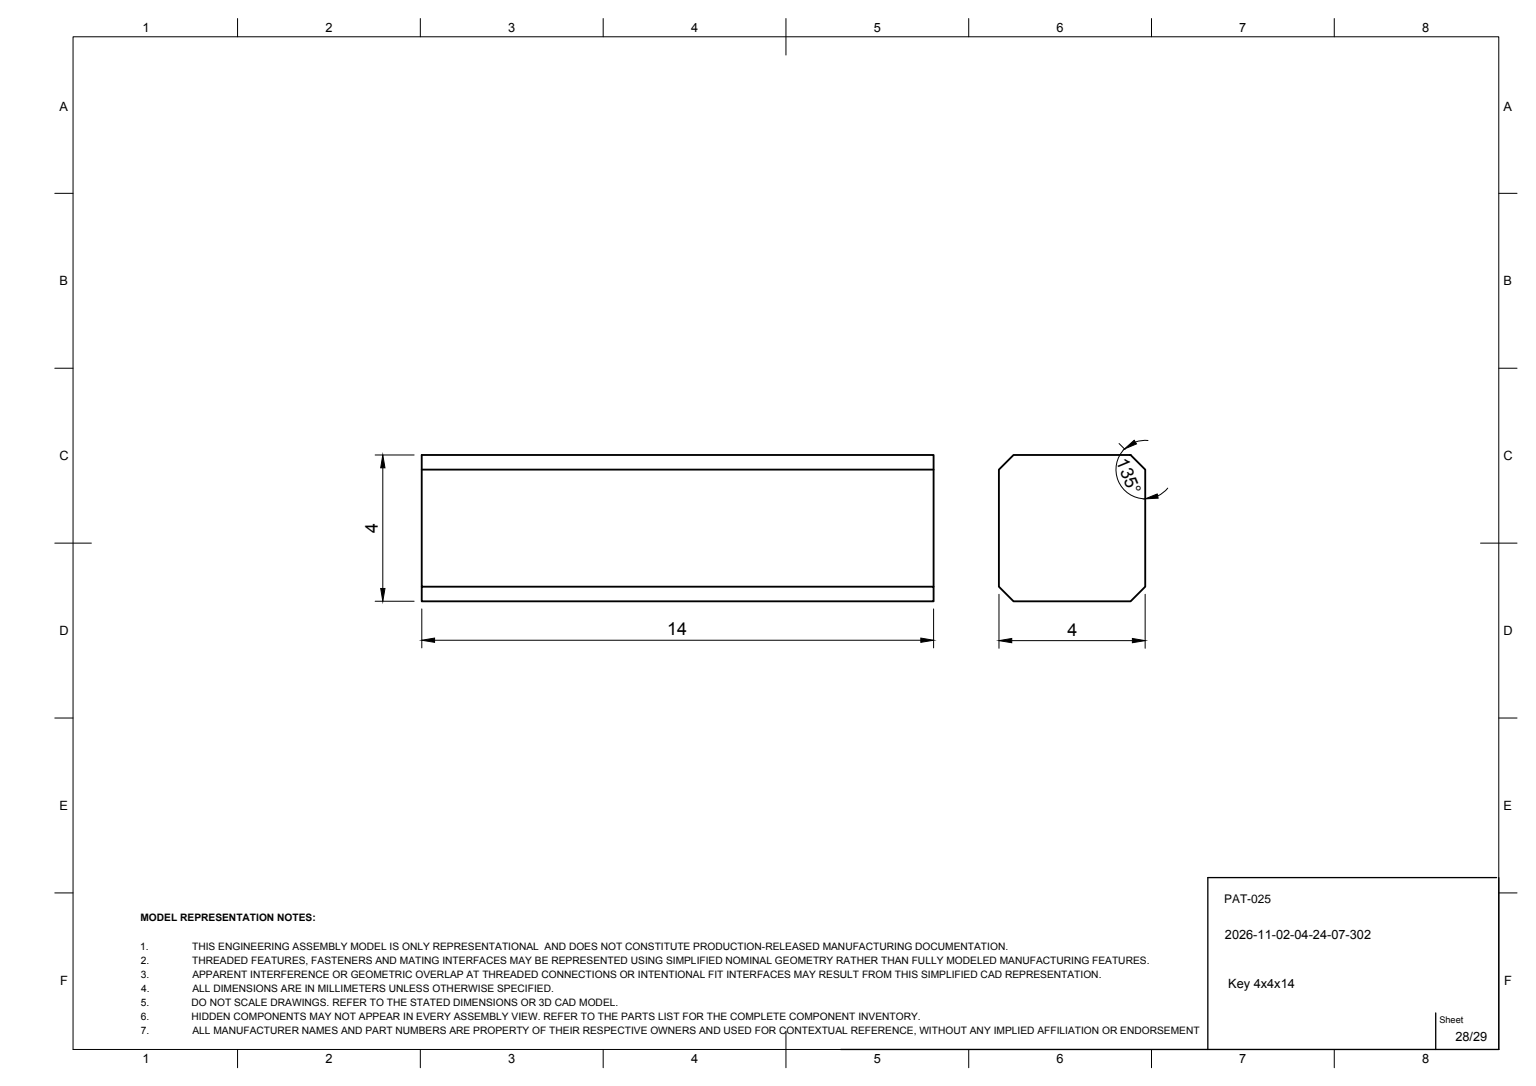
ISO-10303-21;
HEADER;
/* Generated by software containing ST-Developer
 * from STEP Tools, Inc. (www.steptools.com) 
 */

FILE_DESCRIPTION(
/* description */ ('Counter shaft with two pulleys and keyed hub'),
/* implementation_level */ '2;1');

FILE_NAME(
/* name */ 'Key 4x4x14.step',
/* time_stamp */ '2026-10-27T10:46:10-07:00',
/* author */ (''),
/* organization */ (''),
/* preprocessor_version */ 'ST-DEVELOPER v20.2',
/* originating_system */ 'Autodesk Translation Framework v15.17.0.0',
/* authorisation */ '');

FILE_SCHEMA (('AUTOMOTIVE_DESIGN { 1 0 10303 214 3 1 1 }'));
ENDSEC;

DATA;
#10=MECHANICAL_DESIGN_GEOMETRIC_PRESENTATION_REPRESENTATION('',(#312),#10821);
#261=SHAPE_REPRESENTATION_RELATIONSHIP('SRR','None',#10949,#286);
#286=ADVANCED_BREP_SHAPE_REPRESENTATION('',(#337),#10817);
#312=STYLED_ITEM('',(#11135),#337);
#337=MANIFOLD_SOLID_BREP('Body1',#5596);
#548=PLANE('',#6474);
#549=PLANE('',#6475);
#550=PLANE('',#6476);
#551=PLANE('',#6477);
#552=PLANE('',#6478);
#553=PLANE('',#6479);
#554=PLANE('',#6480);
#555=PLANE('',#6481);
#556=PLANE('',#6482);
#557=PLANE('',#6483);
#853=FACE_OUTER_BOUND('',#1256,.T.);
#854=FACE_OUTER_BOUND('',#1257,.T.);
#855=FACE_OUTER_BOUND('',#1258,.T.);
#856=FACE_OUTER_BOUND('',#1259,.T.);
#857=FACE_OUTER_BOUND('',#1260,.T.);
#858=FACE_OUTER_BOUND('',#1261,.T.);
#859=FACE_OUTER_BOUND('',#1262,.T.);
#860=FACE_OUTER_BOUND('',#1263,.T.);
#861=FACE_OUTER_BOUND('',#1264,.T.);
#862=FACE_OUTER_BOUND('',#1265,.T.);
#1256=EDGE_LOOP('',(#4903,#4904,#4905,#4906,#4907,#4908,#4909,#4910));
#1257=EDGE_LOOP('',(#4911,#4912,#4913,#4914));
#1258=EDGE_LOOP('',(#4915,#4916,#4917,#4918));
#1259=EDGE_LOOP('',(#4919,#4920,#4921,#4922));
#1260=EDGE_LOOP('',(#4923,#4924,#4925,#4926));
#1261=EDGE_LOOP('',(#4927,#4928,#4929,#4930,#4931,#4932,#4933,#4934));
#1262=EDGE_LOOP('',(#4935,#4936,#4937,#4938));
#1263=EDGE_LOOP('',(#4939,#4940,#4941,#4942));
#1264=EDGE_LOOP('',(#4943,#4944,#4945,#4946));
#1265=EDGE_LOOP('',(#4947,#4948,#4949,#4950));
#1603=LINE('',#10519,#1992);
#1604=LINE('',#10521,#1993);
#1605=LINE('',#10523,#1994);
#1606=LINE('',#10525,#1995);
#1607=LINE('',#10527,#1996);
#1608=LINE('',#10529,#1997);
#1609=LINE('',#10531,#1998);
#1610=LINE('',#10532,#1999);
#1611=LINE('',#10535,#2000);
#1612=LINE('',#10537,#2001);
#1613=LINE('',#10538,#2002);
#1614=LINE('',#10541,#2003);
#1615=LINE('',#10542,#2004);
#1616=LINE('',#10545,#2005);
#1617=LINE('',#10546,#2006);
#1618=LINE('',#10549,#2007);
#1619=LINE('',#10550,#2008);
#1620=LINE('',#10553,#2009);
#1621=LINE('',#10555,#2010);
#1622=LINE('',#10557,#2011);
#1623=LINE('',#10558,#2012);
#1624=LINE('',#10560,#2013);
#1625=LINE('',#10562,#2014);
#1626=LINE('',#10564,#2015);
#1992=VECTOR('',#8051,1.);
#1993=VECTOR('',#8052,1.);
#1994=VECTOR('',#8053,1.);
#1995=VECTOR('',#8054,1.);
#1996=VECTOR('',#8055,1.);
#1997=VECTOR('',#8056,1.);
#1998=VECTOR('',#8057,1.);
#1999=VECTOR('',#8058,1.);
#2000=VECTOR('',#8061,1.);
#2001=VECTOR('',#8062,1.);
#2002=VECTOR('',#8063,1.);
#2003=VECTOR('',#8066,1.);
#2004=VECTOR('',#8067,1.);
#2005=VECTOR('',#8070,1.);
#2006=VECTOR('',#8071,1.);
#2007=VECTOR('',#8074,1.);
#2008=VECTOR('',#8075,1.);
#2009=VECTOR('',#8078,1.);
#2010=VECTOR('',#8079,1.);
#2011=VECTOR('',#8080,1.);
#2012=VECTOR('',#8081,1.);
#2013=VECTOR('',#8084,1.);
#2014=VECTOR('',#8087,1.);
#2015=VECTOR('',#8090,1.);
#2819=VERTEX_POINT('',#10517);
#2820=VERTEX_POINT('',#10518);
#2821=VERTEX_POINT('',#10520);
#2822=VERTEX_POINT('',#10522);
#2823=VERTEX_POINT('',#10524);
#2824=VERTEX_POINT('',#10526);
#2825=VERTEX_POINT('',#10528);
#2826=VERTEX_POINT('',#10530);
#2827=VERTEX_POINT('',#10534);
#2828=VERTEX_POINT('',#10536);
#2829=VERTEX_POINT('',#10540);
#2830=VERTEX_POINT('',#10544);
#2831=VERTEX_POINT('',#10548);
#2832=VERTEX_POINT('',#10552);
#2833=VERTEX_POINT('',#10554);
#2834=VERTEX_POINT('',#10556);
#3524=EDGE_CURVE('',#2819,#2820,#1603,.T.);
#3525=EDGE_CURVE('',#2821,#2819,#1604,.T.);
#3526=EDGE_CURVE('',#2822,#2821,#1605,.T.);
#3527=EDGE_CURVE('',#2823,#2822,#1606,.T.);
#3528=EDGE_CURVE('',#2824,#2823,#1607,.T.);
#3529=EDGE_CURVE('',#2825,#2824,#1608,.T.);
#3530=EDGE_CURVE('',#2826,#2825,#1609,.T.);
#3531=EDGE_CURVE('',#2820,#2826,#1610,.T.);
#3532=EDGE_CURVE('',#2823,#2827,#1611,.T.);
#3533=EDGE_CURVE('',#2827,#2828,#1612,.T.);
#3534=EDGE_CURVE('',#2828,#2824,#1613,.T.);
#3535=EDGE_CURVE('',#2829,#2822,#1614,.T.);
#3536=EDGE_CURVE('',#2829,#2827,#1615,.T.);
#3537=EDGE_CURVE('',#2821,#2830,#1616,.T.);
#3538=EDGE_CURVE('',#2830,#2829,#1617,.T.);
#3539=EDGE_CURVE('',#2831,#2819,#1618,.T.);
#3540=EDGE_CURVE('',#2831,#2830,#1619,.T.);
#3541=EDGE_CURVE('',#2832,#2831,#1620,.T.);
#3542=EDGE_CURVE('',#2833,#2832,#1621,.T.);
#3543=EDGE_CURVE('',#2834,#2833,#1622,.T.);
#3544=EDGE_CURVE('',#2828,#2834,#1623,.T.);
#3545=EDGE_CURVE('',#2820,#2832,#1624,.T.);
#3546=EDGE_CURVE('',#2833,#2826,#1625,.T.);
#3547=EDGE_CURVE('',#2825,#2834,#1626,.T.);
#4903=ORIENTED_EDGE('',*,*,#3524,.F.);
#4904=ORIENTED_EDGE('',*,*,#3525,.F.);
#4905=ORIENTED_EDGE('',*,*,#3526,.F.);
#4906=ORIENTED_EDGE('',*,*,#3527,.F.);
#4907=ORIENTED_EDGE('',*,*,#3528,.F.);
#4908=ORIENTED_EDGE('',*,*,#3529,.F.);
#4909=ORIENTED_EDGE('',*,*,#3530,.F.);
#4910=ORIENTED_EDGE('',*,*,#3531,.F.);
#4911=ORIENTED_EDGE('',*,*,#3528,.T.);
#4912=ORIENTED_EDGE('',*,*,#3532,.T.);
#4913=ORIENTED_EDGE('',*,*,#3533,.T.);
#4914=ORIENTED_EDGE('',*,*,#3534,.T.);
#4915=ORIENTED_EDGE('',*,*,#3527,.T.);
#4916=ORIENTED_EDGE('',*,*,#3535,.F.);
#4917=ORIENTED_EDGE('',*,*,#3536,.T.);
#4918=ORIENTED_EDGE('',*,*,#3532,.F.);
#4919=ORIENTED_EDGE('',*,*,#3526,.T.);
#4920=ORIENTED_EDGE('',*,*,#3537,.T.);
#4921=ORIENTED_EDGE('',*,*,#3538,.T.);
#4922=ORIENTED_EDGE('',*,*,#3535,.T.);
#4923=ORIENTED_EDGE('',*,*,#3525,.T.);
#4924=ORIENTED_EDGE('',*,*,#3539,.F.);
#4925=ORIENTED_EDGE('',*,*,#3540,.T.);
#4926=ORIENTED_EDGE('',*,*,#3537,.F.);
#4927=ORIENTED_EDGE('',*,*,#3533,.F.);
#4928=ORIENTED_EDGE('',*,*,#3536,.F.);
#4929=ORIENTED_EDGE('',*,*,#3538,.F.);
#4930=ORIENTED_EDGE('',*,*,#3540,.F.);
#4931=ORIENTED_EDGE('',*,*,#3541,.F.);
#4932=ORIENTED_EDGE('',*,*,#3542,.F.);
#4933=ORIENTED_EDGE('',*,*,#3543,.F.);
#4934=ORIENTED_EDGE('',*,*,#3544,.F.);
#4935=ORIENTED_EDGE('',*,*,#3524,.T.);
#4936=ORIENTED_EDGE('',*,*,#3545,.T.);
#4937=ORIENTED_EDGE('',*,*,#3541,.T.);
#4938=ORIENTED_EDGE('',*,*,#3539,.T.);
#4939=ORIENTED_EDGE('',*,*,#3531,.T.);
#4940=ORIENTED_EDGE('',*,*,#3546,.F.);
#4941=ORIENTED_EDGE('',*,*,#3542,.T.);
#4942=ORIENTED_EDGE('',*,*,#3545,.F.);
#4943=ORIENTED_EDGE('',*,*,#3530,.T.);
#4944=ORIENTED_EDGE('',*,*,#3547,.T.);
#4945=ORIENTED_EDGE('',*,*,#3543,.T.);
#4946=ORIENTED_EDGE('',*,*,#3546,.T.);
#4947=ORIENTED_EDGE('',*,*,#3529,.T.);
#4948=ORIENTED_EDGE('',*,*,#3534,.F.);
#4949=ORIENTED_EDGE('',*,*,#3544,.T.);
#4950=ORIENTED_EDGE('',*,*,#3547,.F.);
#5524=ADVANCED_FACE('',(#853),#548,.T.);
#5525=ADVANCED_FACE('',(#854),#549,.T.);
#5526=ADVANCED_FACE('',(#855),#550,.T.);
#5527=ADVANCED_FACE('',(#856),#551,.T.);
#5528=ADVANCED_FACE('',(#857),#552,.T.);
#5529=ADVANCED_FACE('',(#858),#553,.F.);
#5530=ADVANCED_FACE('',(#859),#554,.T.);
#5531=ADVANCED_FACE('',(#860),#555,.T.);
#5532=ADVANCED_FACE('',(#861),#556,.T.);
#5533=ADVANCED_FACE('',(#862),#557,.F.);
#5596=CLOSED_SHELL('',(#5524,#5525,#5526,#5527,#5528,#5529,#5530,#5531,
#5532,#5533));
#6473=AXIS2_PLACEMENT_3D('',#10515,#8047,#8048);
#6474=AXIS2_PLACEMENT_3D('',#10516,#8049,#8050);
#6475=AXIS2_PLACEMENT_3D('',#10533,#8059,#8060);
#6476=AXIS2_PLACEMENT_3D('',#10539,#8064,#8065);
#6477=AXIS2_PLACEMENT_3D('',#10543,#8068,#8069);
#6478=AXIS2_PLACEMENT_3D('',#10547,#8072,#8073);
#6479=AXIS2_PLACEMENT_3D('',#10551,#8076,#8077);
#6480=AXIS2_PLACEMENT_3D('',#10559,#8082,#8083);
#6481=AXIS2_PLACEMENT_3D('',#10561,#8085,#8086);
#6482=AXIS2_PLACEMENT_3D('',#10563,#8088,#8089);
#6483=AXIS2_PLACEMENT_3D('',#10565,#8091,#8092);
#8047=DIRECTION('axis',(0.,0.,1.));
#8048=DIRECTION('refdir',(1.,0.,0.));
#8049=DIRECTION('center_axis',(1.,0.,0.));
#8050=DIRECTION('ref_axis',(0.,0.,-1.));
#8051=DIRECTION('',(0.,0.707106781186547,-0.707106781186548));
#8052=DIRECTION('',(0.,1.,0.));
#8053=DIRECTION('',(0.,0.707106781186547,0.707106781186548));
#8054=DIRECTION('',(0.,0.,1.));
#8055=DIRECTION('',(0.,-0.707106781186548,0.707106781186548));
#8056=DIRECTION('',(0.,-1.,0.));
#8057=DIRECTION('',(0.,-0.707106781186548,-0.707106781186548));
#8058=DIRECTION('',(0.,0.,-1.));
#8059=DIRECTION('center_axis',(0.,-0.707106781186548,-0.707106781186548));
#8060=DIRECTION('ref_axis',(-1.,0.,0.));
#8061=DIRECTION('',(-1.,0.,0.));
#8062=DIRECTION('',(0.,0.707106781186548,-0.707106781186548));
#8063=DIRECTION('',(1.,0.,0.));
#8064=DIRECTION('center_axis',(0.,-1.,0.));
#8065=DIRECTION('ref_axis',(1.,0.,0.));
#8066=DIRECTION('',(1.,0.,0.));
#8067=DIRECTION('',(0.,0.,-1.));
#8068=DIRECTION('center_axis',(0.,-0.707106781186548,0.707106781186547));
#8069=DIRECTION('ref_axis',(1.,0.,0.));
#8070=DIRECTION('',(-1.,0.,0.));
#8071=DIRECTION('',(0.,-0.707106781186547,-0.707106781186548));
#8072=DIRECTION('center_axis',(0.,0.,1.));
#8073=DIRECTION('ref_axis',(1.,0.,0.));
#8074=DIRECTION('',(1.,0.,0.));
#8075=DIRECTION('',(0.,-1.,0.));
#8076=DIRECTION('center_axis',(1.,0.,0.));
#8077=DIRECTION('ref_axis',(0.,0.,-1.));
#8078=DIRECTION('',(0.,-0.707106781186547,0.707106781186548));
#8079=DIRECTION('',(0.,0.,1.));
#8080=DIRECTION('',(0.,0.707106781186548,0.707106781186548));
#8081=DIRECTION('',(0.,1.,0.));
#8082=DIRECTION('center_axis',(0.,0.707106781186548,0.707106781186547));
#8083=DIRECTION('ref_axis',(1.,0.,0.));
#8084=DIRECTION('',(-1.,0.,0.));
#8085=DIRECTION('center_axis',(0.,1.,0.));
#8086=DIRECTION('ref_axis',(-1.,0.,0.));
#8087=DIRECTION('',(1.,0.,0.));
#8088=DIRECTION('center_axis',(0.,0.707106781186548,-0.707106781186548));
#8089=DIRECTION('ref_axis',(-1.,0.,0.));
#8090=DIRECTION('',(-1.,0.,0.));
#8091=DIRECTION('center_axis',(0.,0.,1.));
#8092=DIRECTION('ref_axis',(1.,0.,0.));
#10515=CARTESIAN_POINT('',(0.,0.,0.));
#10516=CARTESIAN_POINT('Origin',(0.7,0.,0.25));
#10517=CARTESIAN_POINT('',(0.7,0.16,0.4));
#10518=CARTESIAN_POINT('',(0.7,0.2,0.36));
#10519=CARTESIAN_POINT('',(0.7,0.1675,0.3925));
#10520=CARTESIAN_POINT('',(0.7,-0.16,0.4));
#10521=CARTESIAN_POINT('',(0.7,0.,0.4));
#10522=CARTESIAN_POINT('',(0.7,-0.2,0.36));
#10523=CARTESIAN_POINT('',(0.7,-0.1675,0.3925));
#10524=CARTESIAN_POINT('',(0.7,-0.2,0.04));
#10525=CARTESIAN_POINT('',(0.7,-0.2,0.125));
#10526=CARTESIAN_POINT('',(0.7,-0.16,0.));
#10527=CARTESIAN_POINT('',(0.7,-0.1925,0.0325));
#10528=CARTESIAN_POINT('',(0.7,0.16,0.));
#10529=CARTESIAN_POINT('',(0.7,0.,0.));
#10530=CARTESIAN_POINT('',(0.7,0.2,0.04));
#10531=CARTESIAN_POINT('',(0.7,0.1925,0.0325));
#10532=CARTESIAN_POINT('',(0.7,0.2,0.125));
#10533=CARTESIAN_POINT('Origin',(-0.4,-0.18,0.02));
#10534=CARTESIAN_POINT('',(-0.7,-0.2,0.04));
#10535=CARTESIAN_POINT('',(-0.4,-0.2,0.04));
#10536=CARTESIAN_POINT('',(-0.7,-0.16,0.));
#10537=CARTESIAN_POINT('',(-0.7,-0.1925,0.0325));
#10538=CARTESIAN_POINT('',(-0.4,-0.16,0.));
#10539=CARTESIAN_POINT('Origin',(-0.8,-0.2,0.));
#10540=CARTESIAN_POINT('',(-0.7,-0.2,0.36));
#10541=CARTESIAN_POINT('',(-0.4,-0.2,0.36));
#10542=CARTESIAN_POINT('',(-0.7,-0.2,0.125));
#10543=CARTESIAN_POINT('Origin',(-0.4,-0.18,0.38));
#10544=CARTESIAN_POINT('',(-0.7,-0.16,0.4));
#10545=CARTESIAN_POINT('',(-0.4,-0.16,0.4));
#10546=CARTESIAN_POINT('',(-0.7,-0.1675,0.3925));
#10547=CARTESIAN_POINT('Origin',(0.,0.,0.4));
#10548=CARTESIAN_POINT('',(-0.7,0.16,0.4));
#10549=CARTESIAN_POINT('',(0.4,0.16,0.4));
#10550=CARTESIAN_POINT('',(-0.7,0.,0.4));
#10551=CARTESIAN_POINT('Origin',(-0.7,0.,0.25));
#10552=CARTESIAN_POINT('',(-0.7,0.2,0.36));
#10553=CARTESIAN_POINT('',(-0.7,0.1675,0.3925));
#10554=CARTESIAN_POINT('',(-0.7,0.2,0.04));
#10555=CARTESIAN_POINT('',(-0.7,0.2,0.125));
#10556=CARTESIAN_POINT('',(-0.7,0.16,0.));
#10557=CARTESIAN_POINT('',(-0.7,0.1925,0.0325));
#10558=CARTESIAN_POINT('',(-0.7,0.,0.));
#10559=CARTESIAN_POINT('Origin',(0.4,0.18,0.38));
#10560=CARTESIAN_POINT('',(0.4,0.2,0.36));
#10561=CARTESIAN_POINT('Origin',(0.8,0.2,0.));
#10562=CARTESIAN_POINT('',(0.4,0.2,0.04));
#10563=CARTESIAN_POINT('Origin',(0.4,0.18,0.02));
#10564=CARTESIAN_POINT('',(0.4,0.16,0.));
#10565=CARTESIAN_POINT('Origin',(0.,0.,0.));
#10787=UNCERTAINTY_MEASURE_WITH_UNIT(LENGTH_MEASURE(0.001),#10822,
'DISTANCE_ACCURACY_VALUE',
'Maximum model space distance between geometric entities at asserted c
onnectivities');
#10791=UNCERTAINTY_MEASURE_WITH_UNIT(LENGTH_MEASURE(0.001),#10822,
'DISTANCE_ACCURACY_VALUE',
'Maximum model space distance between geometric entities at asserted c
onnectivities');
#10817=(
GEOMETRIC_REPRESENTATION_CONTEXT(3)
GLOBAL_UNCERTAINTY_ASSIGNED_CONTEXT((#10787))
GLOBAL_UNIT_ASSIGNED_CONTEXT((#10822,#10824,#10825))
REPRESENTATION_CONTEXT('','3D')
);
#10821=(
GEOMETRIC_REPRESENTATION_CONTEXT(3)
GLOBAL_UNCERTAINTY_ASSIGNED_CONTEXT((#10791))
GLOBAL_UNIT_ASSIGNED_CONTEXT((#10822,#10824,#10825))
REPRESENTATION_CONTEXT('','3D')
);
#10822=(
LENGTH_UNIT()
NAMED_UNIT(*)
SI_UNIT(.CENTI.,.METRE.)
);
#10824=(
NAMED_UNIT(*)
PLANE_ANGLE_UNIT()
SI_UNIT($,.RADIAN.)
);
#10825=(
NAMED_UNIT(*)
SI_UNIT($,.STERADIAN.)
SOLID_ANGLE_UNIT()
);
#10851=SHAPE_DEFINITION_REPRESENTATION(#10899,#10949);
#10899=PRODUCT_DEFINITION_SHAPE('',$,#10979);
#10949=SHAPE_REPRESENTATION('',(#6473),#10817);
#10953=PRODUCT_DEFINITION_CONTEXT('part definition',#11042,'design');
#10979=PRODUCT_DEFINITION('Key 4x4x14','Key 4x4x14',#11008,#10953);
#11008=PRODUCT_DEFINITION_FORMATION('',$,#11069);
#11042=APPLICATION_CONTEXT(
'Core Data for Automotive Mechanical Design Process');
#11043=PRODUCT_CONTEXT('part definition',#11042,'mechanical');
#11069=PRODUCT('Key 4x4x14','Key 4x4x14','Key 4x4x14',(#11043));
#11129=COLOUR_RGB('Grey',0.48,0.52,0.57);
#11130=FILL_AREA_STYLE_COLOUR('',#11129);
#11131=FILL_AREA_STYLE('',(#11130));
#11132=SURFACE_STYLE_FILL_AREA(#11131);
#11133=SURFACE_SIDE_STYLE('',(#11132));
#11134=SURFACE_STYLE_USAGE(.BOTH.,#11133);
#11135=PRESENTATION_STYLE_ASSIGNMENT((#11134));
ENDSEC;
END-ISO-10303-21;
